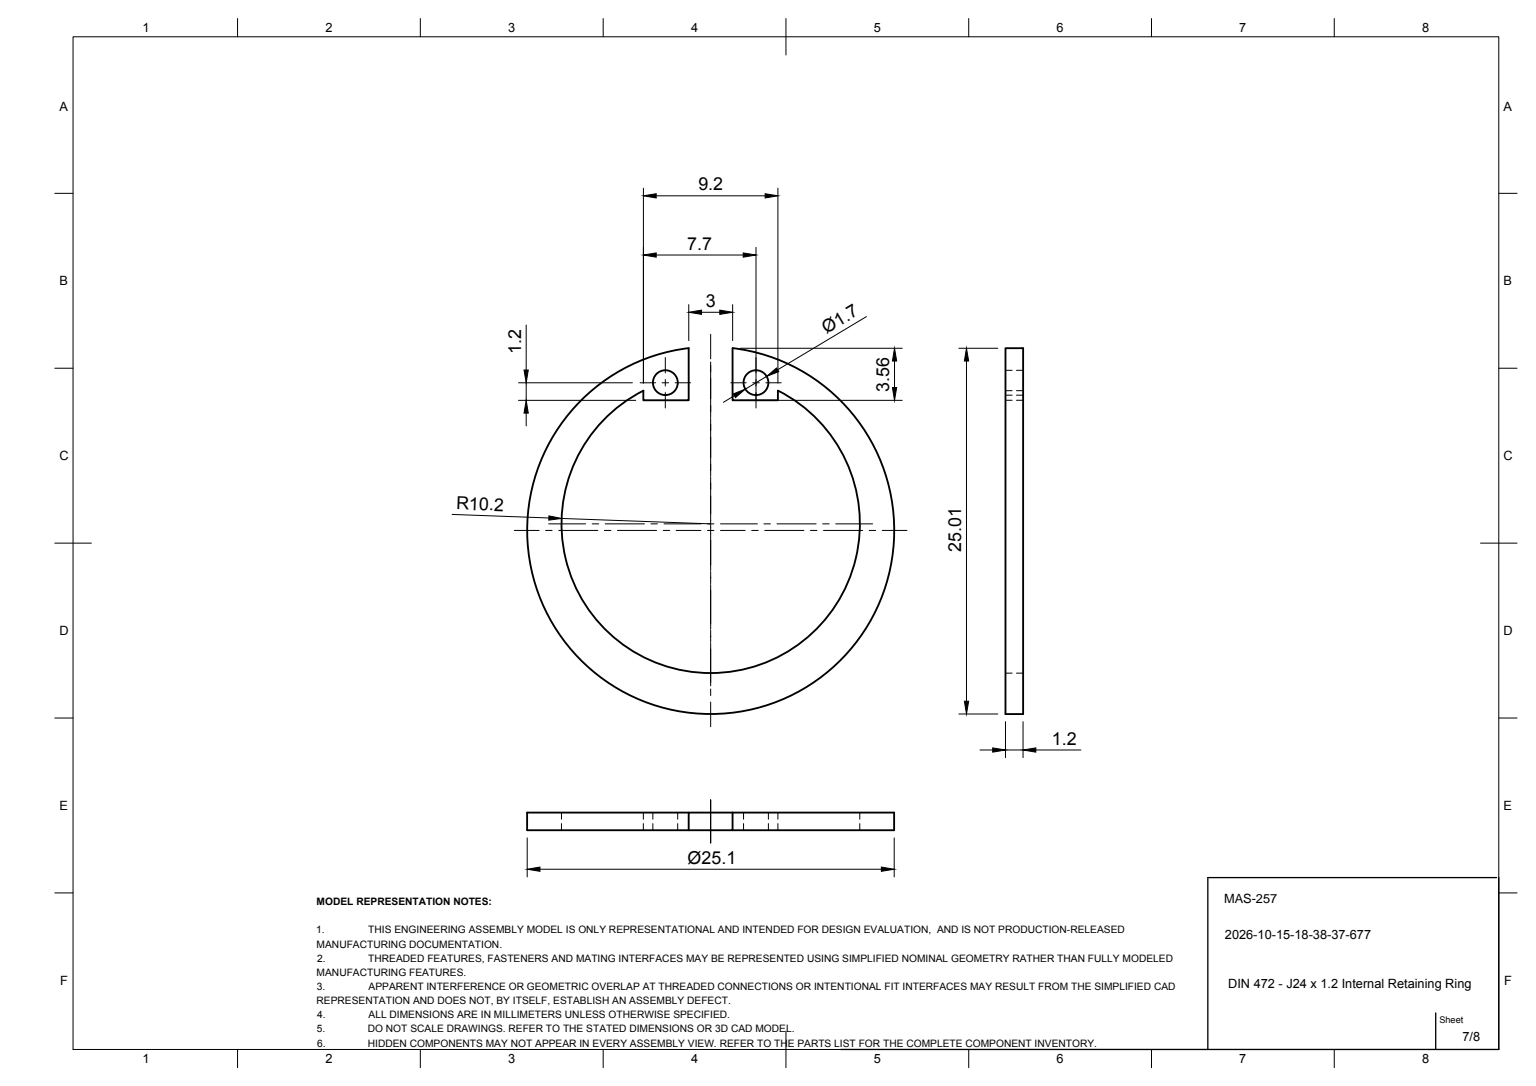
ISO-10303-21;
HEADER;
FILE_DESCRIPTION((''),'2;1');
FILE_NAME('DIN 472 - J24 x 1.2 Internal Retaining Ring.step','2026-10-05T22:33:56+05:00',(''),(''),'','','');
FILE_SCHEMA (('AUTOMOTIVE_DESIGN { 1 0 10303 214 3 1 1 }'));
ENDSEC;
DATA;
#10=MECHANICAL_DESIGN_GEOMETRIC_PRESENTATION_REPRESENTATION('',(#435),#16942);
#421=SHAPE_REPRESENTATION_RELATIONSHIP('SRR','None',#17025,#428) ;
#428=ADVANCED_BREP_SHAPE_REPRESENTATION('',(#442),#16941) ;
#435=STYLED_ITEM('',(#17069),#442) ;
#442=MANIFOLD_SOLID_BREP('DIN 472 - J24 x 1.2 Internal Retaining Ring',
#8184) ;
#733=FACE_BOUND('',#1985,.T.) ;
#734=FACE_BOUND('',#1986,.T.) ;
#735=FACE_BOUND('',#1994,.T.) ;
#736=FACE_BOUND('',#1995,.T.) ;
#969=PLANE('',#8900) ;
#970=PLANE('',#8901) ;
#971=PLANE('',#8902) ;
#972=PLANE('',#8903) ;
#973=PLANE('',#8909) ;
#974=PLANE('',#8910) ;
#975=PLANE('',#8913) ;
#976=PLANE('',#8916) ;
#1057=CYLINDRICAL_SURFACE('',#8897,0.85) ;
#1058=CYLINDRICAL_SURFACE('',#8907,0.85) ;
#1059=CYLINDRICAL_SURFACE('',#8911,10.2) ;
#1060=CYLINDRICAL_SURFACE('',#8914,12.55) ;
#1491=FACE_OUTER_BOUND('',#1980,.T.) ;
#1492=FACE_OUTER_BOUND('',#1981,.T.) ;
#1493=FACE_OUTER_BOUND('',#1982,.T.) ;
#1494=FACE_OUTER_BOUND('',#1983,.T.) ;
#1495=FACE_OUTER_BOUND('',#1984,.T.) ;
#1496=FACE_OUTER_BOUND('',#1987,.T.) ;
#1497=FACE_OUTER_BOUND('',#1988,.T.) ;
#1498=FACE_OUTER_BOUND('',#1989,.T.) ;
#1499=FACE_OUTER_BOUND('',#1990,.T.) ;
#1500=FACE_OUTER_BOUND('',#1991,.T.) ;
#1501=FACE_OUTER_BOUND('',#1992,.T.) ;
#1502=FACE_OUTER_BOUND('',#1993,.T.) ;
#1980=EDGE_LOOP('',(#7647,#7648,#7649,#7650)) ;
#1981=EDGE_LOOP('',(#7651,#7652,#7653,#7654)) ;
#1982=EDGE_LOOP('',(#7655,#7656,#7657,#7658)) ;
#1983=EDGE_LOOP('',(#7659,#7660,#7661,#7662)) ;
#1984=EDGE_LOOP('',(#7663,#7664,#7665,#7666,#7667,#7668,#7669,#7670)) ;
#1985=EDGE_LOOP('',(#7671)) ;
#1986=EDGE_LOOP('',(#7672)) ;
#1987=EDGE_LOOP('',(#7673,#7674,#7675,#7676)) ;
#1988=EDGE_LOOP('',(#7677,#7678,#7679,#7680)) ;
#1989=EDGE_LOOP('',(#7681,#7682,#7683,#7684)) ;
#1990=EDGE_LOOP('',(#7685,#7686,#7687,#7688)) ;
#1991=EDGE_LOOP('',(#7689,#7690,#7691,#7692)) ;
#1992=EDGE_LOOP('',(#7693,#7694,#7695,#7696)) ;
#1993=EDGE_LOOP('',(#7697,#7698,#7699,#7700,#7701,#7702,#7703,#7704)) ;
#1994=EDGE_LOOP('',(#7705)) ;
#1995=EDGE_LOOP('',(#7706)) ;
#2536=LINE('',#16812,#3098) ;
#2537=LINE('',#16817,#3099) ;
#2538=LINE('',#16819,#3100) ;
#2539=LINE('',#16821,#3101) ;
#2540=LINE('',#16822,#3102) ;
#2541=LINE('',#16825,#3103) ;
#2542=LINE('',#16827,#3104) ;
#2543=LINE('',#16828,#3105) ;
#2544=LINE('',#16831,#3106) ;
#2545=LINE('',#16833,#3107) ;
#2546=LINE('',#16834,#3108) ;
#2547=LINE('',#16839,#3109) ;
#2548=LINE('',#16841,#3110) ;
#2549=LINE('',#16843,#3111) ;
#2550=LINE('',#16850,#3112) ;
#2551=LINE('',#16853,#3113) ;
#2552=LINE('',#16855,#3114) ;
#2553=LINE('',#16856,#3115) ;
#2554=LINE('',#16859,#3116) ;
#2555=LINE('',#16860,#3117) ;
#2556=LINE('',#16865,#3118) ;
#2557=LINE('',#16866,#3119) ;
#3098=VECTOR('',#10784,0.85) ;
#3099=VECTOR('',#10789,10.) ;
#3100=VECTOR('',#10790,10.) ;
#3101=VECTOR('',#10791,10.) ;
#3102=VECTOR('',#10792,10.) ;
#3103=VECTOR('',#10795,10.) ;
#3104=VECTOR('',#10796,10.) ;
#3105=VECTOR('',#10797,10.) ;
#3106=VECTOR('',#10800,10.) ;
#3107=VECTOR('',#10801,10.) ;
#3108=VECTOR('',#10802,10.) ;
#3109=VECTOR('',#10807,10.) ;
#3110=VECTOR('',#10808,10.) ;
#3111=VECTOR('',#10809,10.) ;
#3112=VECTOR('',#10818,0.85) ;
#3113=VECTOR('',#10821,10.) ;
#3114=VECTOR('',#10822,10.) ;
#3115=VECTOR('',#10823,10.) ;
#3116=VECTOR('',#10826,10.) ;
#3117=VECTOR('',#10827,10.) ;
#3118=VECTOR('',#10834,10.) ;
#3119=VECTOR('',#10835,10.) ;
#3390=CIRCLE('',#8898,0.85) ;
#3391=CIRCLE('',#8899,0.85) ;
#3392=CIRCLE('',#8904,10.2) ;
#3393=CIRCLE('',#8905,12.55) ;
#3394=CIRCLE('',#8906,0.85) ;
#3395=CIRCLE('',#8908,0.85) ;
#3396=CIRCLE('',#8912,10.2) ;
#3397=CIRCLE('',#8915,12.55) ;
#4153=VERTEX_POINT('',#16809) ;
#4154=VERTEX_POINT('',#16811) ;
#4155=VERTEX_POINT('',#16815) ;
#4156=VERTEX_POINT('',#16816) ;
#4157=VERTEX_POINT('',#16818) ;
#4158=VERTEX_POINT('',#16820) ;
#4159=VERTEX_POINT('',#16824) ;
#4160=VERTEX_POINT('',#16826) ;
#4161=VERTEX_POINT('',#16830) ;
#4162=VERTEX_POINT('',#16832) ;
#4163=VERTEX_POINT('',#16836) ;
#4164=VERTEX_POINT('',#16838) ;
#4165=VERTEX_POINT('',#16840) ;
#4166=VERTEX_POINT('',#16842) ;
#4167=VERTEX_POINT('',#16845) ;
#4168=VERTEX_POINT('',#16848) ;
#4169=VERTEX_POINT('',#16852) ;
#4170=VERTEX_POINT('',#16854) ;
#4171=VERTEX_POINT('',#16858) ;
#4172=VERTEX_POINT('',#16864) ;
#5321=EDGE_CURVE('',#4153,#4153,#3390,.T.) ;
#5322=EDGE_CURVE('',#4153,#4154,#2536,.T.) ;
#5323=EDGE_CURVE('',#4154,#4154,#3391,.T.) ;
#5324=EDGE_CURVE('',#4155,#4156,#2537,.T.) ;
#5325=EDGE_CURVE('',#4157,#4155,#2538,.T.) ;
#5326=EDGE_CURVE('',#4158,#4157,#2539,.T.) ;
#5327=EDGE_CURVE('',#4156,#4158,#2540,.T.) ;
#5328=EDGE_CURVE('',#4158,#4159,#2541,.T.) ;
#5329=EDGE_CURVE('',#4160,#4157,#2542,.T.) ;
#5330=EDGE_CURVE('',#4159,#4160,#2543,.T.) ;
#5331=EDGE_CURVE('',#4161,#4160,#2544,.T.) ;
#5332=EDGE_CURVE('',#4162,#4161,#2545,.T.) ;
#5333=EDGE_CURVE('',#4159,#4162,#2546,.T.) ;
#5334=EDGE_CURVE('',#4155,#4163,#3392,.T.) ;
#5335=EDGE_CURVE('',#4163,#4164,#2547,.T.) ;
#5336=EDGE_CURVE('',#4164,#4165,#2548,.T.) ;
#5337=EDGE_CURVE('',#4165,#4166,#2549,.T.) ;
#5338=EDGE_CURVE('',#4166,#4161,#3393,.T.) ;
#5339=EDGE_CURVE('',#4167,#4167,#3394,.T.) ;
#5340=EDGE_CURVE('',#4168,#4168,#3395,.T.) ;
#5341=EDGE_CURVE('',#4168,#4167,#2550,.T.) ;
#5342=EDGE_CURVE('',#4169,#4163,#2551,.T.) ;
#5343=EDGE_CURVE('',#4169,#4170,#2552,.T.) ;
#5344=EDGE_CURVE('',#4170,#4164,#2553,.T.) ;
#5345=EDGE_CURVE('',#4170,#4171,#2554,.T.) ;
#5346=EDGE_CURVE('',#4171,#4165,#2555,.T.) ;
#5347=EDGE_CURVE('',#4156,#4169,#3396,.T.) ;
#5348=EDGE_CURVE('',#4172,#4171,#2556,.T.) ;
#5349=EDGE_CURVE('',#4166,#4172,#2557,.T.) ;
#5350=EDGE_CURVE('',#4172,#4162,#3397,.T.) ;
#7647=ORIENTED_EDGE('',*,*,#5321,.F.) ;
#7648=ORIENTED_EDGE('',*,*,#5322,.T.) ;
#7649=ORIENTED_EDGE('',*,*,#5323,.F.) ;
#7650=ORIENTED_EDGE('',*,*,#5322,.F.) ;
#7651=ORIENTED_EDGE('',*,*,#5324,.F.) ;
#7652=ORIENTED_EDGE('',*,*,#5325,.F.) ;
#7653=ORIENTED_EDGE('',*,*,#5326,.F.) ;
#7654=ORIENTED_EDGE('',*,*,#5327,.F.) ;
#7655=ORIENTED_EDGE('',*,*,#5328,.F.) ;
#7656=ORIENTED_EDGE('',*,*,#5326,.T.) ;
#7657=ORIENTED_EDGE('',*,*,#5329,.F.) ;
#7658=ORIENTED_EDGE('',*,*,#5330,.F.) ;
#7659=ORIENTED_EDGE('',*,*,#5331,.F.) ;
#7660=ORIENTED_EDGE('',*,*,#5332,.F.) ;
#7661=ORIENTED_EDGE('',*,*,#5333,.F.) ;
#7662=ORIENTED_EDGE('',*,*,#5330,.T.) ;
#7663=ORIENTED_EDGE('',*,*,#5331,.T.) ;
#7664=ORIENTED_EDGE('',*,*,#5329,.T.) ;
#7665=ORIENTED_EDGE('',*,*,#5325,.T.) ;
#7666=ORIENTED_EDGE('',*,*,#5334,.T.) ;
#7667=ORIENTED_EDGE('',*,*,#5335,.T.) ;
#7668=ORIENTED_EDGE('',*,*,#5336,.T.) ;
#7669=ORIENTED_EDGE('',*,*,#5337,.T.) ;
#7670=ORIENTED_EDGE('',*,*,#5338,.T.) ;
#7671=ORIENTED_EDGE('',*,*,#5323,.T.) ;
#7672=ORIENTED_EDGE('',*,*,#5339,.T.) ;
#7673=ORIENTED_EDGE('',*,*,#5340,.F.) ;
#7674=ORIENTED_EDGE('',*,*,#5341,.T.) ;
#7675=ORIENTED_EDGE('',*,*,#5339,.F.) ;
#7676=ORIENTED_EDGE('',*,*,#5341,.F.) ;
#7677=ORIENTED_EDGE('',*,*,#5342,.F.) ;
#7678=ORIENTED_EDGE('',*,*,#5343,.T.) ;
#7679=ORIENTED_EDGE('',*,*,#5344,.T.) ;
#7680=ORIENTED_EDGE('',*,*,#5335,.F.) ;
#7681=ORIENTED_EDGE('',*,*,#5345,.T.) ;
#7682=ORIENTED_EDGE('',*,*,#5346,.T.) ;
#7683=ORIENTED_EDGE('',*,*,#5336,.F.) ;
#7684=ORIENTED_EDGE('',*,*,#5344,.F.) ;
#7685=ORIENTED_EDGE('',*,*,#5324,.T.) ;
#7686=ORIENTED_EDGE('',*,*,#5347,.T.) ;
#7687=ORIENTED_EDGE('',*,*,#5342,.T.) ;
#7688=ORIENTED_EDGE('',*,*,#5334,.F.) ;
#7689=ORIENTED_EDGE('',*,*,#5348,.F.) ;
#7690=ORIENTED_EDGE('',*,*,#5349,.F.) ;
#7691=ORIENTED_EDGE('',*,*,#5337,.F.) ;
#7692=ORIENTED_EDGE('',*,*,#5346,.F.) ;
#7693=ORIENTED_EDGE('',*,*,#5349,.T.) ;
#7694=ORIENTED_EDGE('',*,*,#5350,.T.) ;
#7695=ORIENTED_EDGE('',*,*,#5332,.T.) ;
#7696=ORIENTED_EDGE('',*,*,#5338,.F.) ;
#7697=ORIENTED_EDGE('',*,*,#5333,.T.) ;
#7698=ORIENTED_EDGE('',*,*,#5350,.F.) ;
#7699=ORIENTED_EDGE('',*,*,#5348,.T.) ;
#7700=ORIENTED_EDGE('',*,*,#5345,.F.) ;
#7701=ORIENTED_EDGE('',*,*,#5343,.F.) ;
#7702=ORIENTED_EDGE('',*,*,#5347,.F.) ;
#7703=ORIENTED_EDGE('',*,*,#5327,.T.) ;
#7704=ORIENTED_EDGE('',*,*,#5328,.T.) ;
#7705=ORIENTED_EDGE('',*,*,#5321,.T.) ;
#7706=ORIENTED_EDGE('',*,*,#5340,.T.) ;
#8166=ADVANCED_FACE('',(#1491),#1057,.F.) ;
#8167=ADVANCED_FACE('',(#1492),#969,.T.) ;
#8168=ADVANCED_FACE('',(#1493),#970,.T.) ;
#8169=ADVANCED_FACE('',(#1494),#971,.F.) ;
#8170=ADVANCED_FACE('',(#1495,#733,#734),#972,.T.) ;
#8171=ADVANCED_FACE('',(#1496),#1058,.F.) ;
#8172=ADVANCED_FACE('',(#1497),#973,.T.) ;
#8173=ADVANCED_FACE('',(#1498),#974,.T.) ;
#8174=ADVANCED_FACE('',(#1499),#1059,.F.) ;
#8175=ADVANCED_FACE('',(#1500),#975,.F.) ;
#8176=ADVANCED_FACE('',(#1501),#1060,.T.) ;
#8177=ADVANCED_FACE('',(#1502,#735,#736),#976,.F.) ;
#8184=CLOSED_SHELL('',(#8166,#8167,#8168,#8169,#8170,#8171,#8172,#8173,
#8174,#8175,#8176,#8177)) ;
#8896=AXIS2_PLACEMENT_3D('',#16807,#10778,#10779) ;
#8897=AXIS2_PLACEMENT_3D('',#16808,#10780,#10781) ;
#8898=AXIS2_PLACEMENT_3D('',#16810,#10782,#10783) ;
#8899=AXIS2_PLACEMENT_3D('',#16813,#10785,#10786) ;
#8900=AXIS2_PLACEMENT_3D('',#16814,#10787,#10788) ;
#8901=AXIS2_PLACEMENT_3D('',#16823,#10793,#10794) ;
#8902=AXIS2_PLACEMENT_3D('',#16829,#10798,#10799) ;
#8903=AXIS2_PLACEMENT_3D('',#16835,#10803,#10804) ;
#8904=AXIS2_PLACEMENT_3D('',#16837,#10805,#10806) ;
#8905=AXIS2_PLACEMENT_3D('',#16844,#10810,#10811) ;
#8906=AXIS2_PLACEMENT_3D('',#16846,#10812,#10813) ;
#8907=AXIS2_PLACEMENT_3D('',#16847,#10814,#10815) ;
#8908=AXIS2_PLACEMENT_3D('',#16849,#10816,#10817) ;
#8909=AXIS2_PLACEMENT_3D('',#16851,#10819,#10820) ;
#8910=AXIS2_PLACEMENT_3D('',#16857,#10824,#10825) ;
#8911=AXIS2_PLACEMENT_3D('',#16861,#10828,#10829) ;
#8912=AXIS2_PLACEMENT_3D('',#16862,#10830,#10831) ;
#8913=AXIS2_PLACEMENT_3D('',#16863,#10832,#10833) ;
#8914=AXIS2_PLACEMENT_3D('',#16867,#10836,#10837) ;
#8915=AXIS2_PLACEMENT_3D('',#16868,#10838,#10839) ;
#8916=AXIS2_PLACEMENT_3D('',#16869,#10840,#10841) ;
#10778=DIRECTION('axis',(0.,0.,1.)) ;
#10779=DIRECTION('refdir',(1.,0.,0.)) ;
#10780=DIRECTION('center_axis',(1.,0.,0.)) ;
#10781=DIRECTION('ref_axis',(0.,0.,-1.)) ;
#10782=DIRECTION('center_axis',(1.,0.,0.)) ;
#10783=DIRECTION('ref_axis',(0.,0.,-1.)) ;
#10784=DIRECTION('',(1.,0.,0.)) ;
#10785=DIRECTION('center_axis',(-1.,0.,0.)) ;
#10786=DIRECTION('ref_axis',(0.,0.,-1.)) ;
#10787=DIRECTION('center_axis',(0.,0.,-1.)) ;
#10788=DIRECTION('ref_axis',(0.,1.,0.)) ;
#10789=DIRECTION('',(-1.,0.,0.)) ;
#10790=DIRECTION('',(0.,1.,0.)) ;
#10791=DIRECTION('',(1.,0.,0.)) ;
#10792=DIRECTION('',(0.,-1.,0.)) ;
#10793=DIRECTION('center_axis',(0.,-1.,0.)) ;
#10794=DIRECTION('ref_axis',(0.,0.,-1.)) ;
#10795=DIRECTION('',(0.,0.,1.)) ;
#10796=DIRECTION('',(0.,0.,-1.)) ;
#10797=DIRECTION('',(1.,0.,0.)) ;
#10798=DIRECTION('center_axis',(0.,0.,-1.)) ;
#10799=DIRECTION('ref_axis',(0.,1.,0.)) ;
#10800=DIRECTION('',(0.,-1.,0.)) ;
#10801=DIRECTION('',(1.,0.,0.)) ;
#10802=DIRECTION('',(0.,1.,0.)) ;
#10803=DIRECTION('center_axis',(1.,0.,0.)) ;
#10804=DIRECTION('ref_axis',(0.,0.,-1.)) ;
#10805=DIRECTION('center_axis',(-1.,0.,0.)) ;
#10806=DIRECTION('ref_axis',(0.,0.,-1.)) ;
#10807=DIRECTION('',(0.,-1.,0.)) ;
#10808=DIRECTION('',(0.,0.,-1.)) ;
#10809=DIRECTION('',(0.,1.,0.)) ;
#10810=DIRECTION('center_axis',(1.,0.,0.)) ;
#10811=DIRECTION('ref_axis',(0.,0.,-1.)) ;
#10812=DIRECTION('center_axis',(-1.,0.,0.)) ;
#10813=DIRECTION('ref_axis',(0.,0.,-1.)) ;
#10814=DIRECTION('center_axis',(1.,0.,0.)) ;
#10815=DIRECTION('ref_axis',(0.,0.,-1.)) ;
#10816=DIRECTION('center_axis',(1.,0.,0.)) ;
#10817=DIRECTION('ref_axis',(0.,0.,-1.)) ;
#10818=DIRECTION('',(1.,0.,0.)) ;
#10819=DIRECTION('center_axis',(0.,0.,1.)) ;
#10820=DIRECTION('ref_axis',(0.,-1.,0.)) ;
#10821=DIRECTION('',(1.,0.,0.)) ;
#10822=DIRECTION('',(0.,-1.,0.)) ;
#10823=DIRECTION('',(1.,0.,0.)) ;
#10824=DIRECTION('center_axis',(0.,-1.,0.)) ;
#10825=DIRECTION('ref_axis',(0.,0.,-1.)) ;
#10826=DIRECTION('',(0.,0.,-1.)) ;
#10827=DIRECTION('',(1.,0.,0.)) ;
#10828=DIRECTION('center_axis',(1.,0.,0.)) ;
#10829=DIRECTION('ref_axis',(0.,-1.,-6.12323399573677E-17)) ;
#10830=DIRECTION('center_axis',(-1.,0.,0.)) ;
#10831=DIRECTION('ref_axis',(0.,0.,-1.)) ;
#10832=DIRECTION('center_axis',(0.,0.,1.)) ;
#10833=DIRECTION('ref_axis',(0.,-1.,0.)) ;
#10834=DIRECTION('',(0.,-1.,0.)) ;
#10835=DIRECTION('',(-1.,0.,0.)) ;
#10836=DIRECTION('center_axis',(1.,0.,0.)) ;
#10837=DIRECTION('ref_axis',(0.,-1.,1.83697019872103E-16)) ;
#10838=DIRECTION('center_axis',(1.,0.,0.)) ;
#10839=DIRECTION('ref_axis',(0.,0.,-1.)) ;
#10840=DIRECTION('center_axis',(1.,0.,0.)) ;
#10841=DIRECTION('ref_axis',(0.,0.,-1.)) ;
#16807=CARTESIAN_POINT('',(0.,0.,0.)) ;
#16808=CARTESIAN_POINT('Origin',(27.85,35.6,22.4)) ;
#16809=CARTESIAN_POINT('',(27.85,35.6,23.25)) ;
#16810=CARTESIAN_POINT('Origin',(27.85,35.6,22.4)) ;
#16811=CARTESIAN_POINT('',(29.05,35.6,23.25)) ;
#16812=CARTESIAN_POINT('',(27.85,35.6,23.25)) ;
#16813=CARTESIAN_POINT('Origin',(29.05,35.6,22.4)) ;
#16814=CARTESIAN_POINT('Origin',(27.85,34.4,20.9)) ;
#16815=CARTESIAN_POINT('',(29.05,35.0538453413928,20.9)) ;
#16816=CARTESIAN_POINT('',(27.85,35.0538453413928,20.9)) ;
#16817=CARTESIAN_POINT('',(27.85,35.0538453413928,20.9)) ;
#16818=CARTESIAN_POINT('',(29.05,34.4,20.9)) ;
#16819=CARTESIAN_POINT('',(29.05,36.4,20.9)) ;
#16820=CARTESIAN_POINT('',(27.85,34.4,20.9)) ;
#16821=CARTESIAN_POINT('',(27.85,34.4,20.9)) ;
#16822=CARTESIAN_POINT('',(27.85,36.4,20.9)) ;
#16823=CARTESIAN_POINT('Origin',(27.85,34.4,24.)) ;
#16824=CARTESIAN_POINT('',(27.85,34.4,24.)) ;
#16825=CARTESIAN_POINT('',(27.85,34.4,20.9)) ;
#16826=CARTESIAN_POINT('',(29.05,34.4,24.)) ;
#16827=CARTESIAN_POINT('',(29.05,34.4,20.9)) ;
#16828=CARTESIAN_POINT('',(27.85,34.4,24.)) ;
#16829=CARTESIAN_POINT('Origin',(27.85,34.5,24.)) ;
#16830=CARTESIAN_POINT('',(29.05,37.9600361155175,24.)) ;
#16831=CARTESIAN_POINT('',(29.05,34.4,24.)) ;
#16832=CARTESIAN_POINT('',(27.85,37.9600361155175,24.)) ;
#16833=CARTESIAN_POINT('',(27.85,37.9600361155175,24.)) ;
#16834=CARTESIAN_POINT('',(27.85,30.,24.)) ;
#16835=CARTESIAN_POINT('Origin',(29.05,25.5,25.5)) ;
#16836=CARTESIAN_POINT('',(29.05,35.0538453413928,30.1)) ;
#16837=CARTESIAN_POINT('Origin',(29.05,25.95,25.5)) ;
#16838=CARTESIAN_POINT('',(29.05,34.4,30.1)) ;
#16839=CARTESIAN_POINT('',(29.05,36.4,30.1)) ;
#16840=CARTESIAN_POINT('',(29.05,34.4,27.)) ;
#16841=CARTESIAN_POINT('',(29.05,34.4,30.1)) ;
#16842=CARTESIAN_POINT('',(29.05,37.9600361155175,27.)) ;
#16843=CARTESIAN_POINT('',(29.05,32.,27.)) ;
#16844=CARTESIAN_POINT('Origin',(29.05,25.5,25.5)) ;
#16845=CARTESIAN_POINT('',(29.05,35.6,29.45)) ;
#16846=CARTESIAN_POINT('Origin',(29.05,35.6,28.6)) ;
#16847=CARTESIAN_POINT('Origin',(27.85,35.6,28.6)) ;
#16848=CARTESIAN_POINT('',(27.85,35.6,29.45)) ;
#16849=CARTESIAN_POINT('Origin',(27.85,35.6,28.6)) ;
#16850=CARTESIAN_POINT('',(27.85,35.6,29.45)) ;
#16851=CARTESIAN_POINT('Origin',(27.85,36.4,30.1)) ;
#16852=CARTESIAN_POINT('',(27.85,35.0538453413928,30.1)) ;
#16853=CARTESIAN_POINT('',(27.85,35.0538453413928,30.1)) ;
#16854=CARTESIAN_POINT('',(27.85,34.4,30.1)) ;
#16855=CARTESIAN_POINT('',(27.85,36.4,30.1)) ;
#16856=CARTESIAN_POINT('',(27.85,34.4,30.1)) ;
#16857=CARTESIAN_POINT('Origin',(27.85,34.4,30.1)) ;
#16858=CARTESIAN_POINT('',(27.85,34.4,27.)) ;
#16859=CARTESIAN_POINT('',(27.85,34.4,30.1)) ;
#16860=CARTESIAN_POINT('',(27.85,34.4,27.)) ;
#16861=CARTESIAN_POINT('Origin',(27.85,25.95,25.5)) ;
#16862=CARTESIAN_POINT('Origin',(27.85,25.95,25.5)) ;
#16863=CARTESIAN_POINT('Origin',(27.85,38.5,27.)) ;
#16864=CARTESIAN_POINT('',(27.85,37.9600361155175,27.)) ;
#16865=CARTESIAN_POINT('',(27.85,32.,27.)) ;
#16866=CARTESIAN_POINT('',(27.85,37.9600361155175,27.)) ;
#16867=CARTESIAN_POINT('Origin',(27.85,25.5,25.5)) ;
#16868=CARTESIAN_POINT('Origin',(27.85,25.5,25.5)) ;
#16869=CARTESIAN_POINT('Origin',(27.85,25.5,25.5)) ;
#16932=UNCERTAINTY_MEASURE_WITH_UNIT(LENGTH_MEASURE(0.01),#16943,
'DISTANCE_ACCURACY_VALUE',
'Maximum model space distance between geometric entities at asserted c
onnectivities') ;
#16933=UNCERTAINTY_MEASURE_WITH_UNIT(LENGTH_MEASURE(0.01),#16943,
'DISTANCE_ACCURACY_VALUE',
'Maximum model space distance between geometric entities at asserted c
onnectivities') ;
#16941=(
GEOMETRIC_REPRESENTATION_CONTEXT(3)
GLOBAL_UNCERTAINTY_ASSIGNED_CONTEXT((#16932))
GLOBAL_UNIT_ASSIGNED_CONTEXT((#16943,#16945,#16946))
REPRESENTATION_CONTEXT('','3D')
) ;
#16942=(
GEOMETRIC_REPRESENTATION_CONTEXT(3)
GLOBAL_UNCERTAINTY_ASSIGNED_CONTEXT((#16933))
GLOBAL_UNIT_ASSIGNED_CONTEXT((#16943,#16945,#16946))
REPRESENTATION_CONTEXT('','3D')
) ;
#16943=(
LENGTH_UNIT()
NAMED_UNIT(*)
SI_UNIT(.MILLI.,.METRE.)
) ;
#16945=(
NAMED_UNIT(*)
PLANE_ANGLE_UNIT()
SI_UNIT($,.RADIAN.)
) ;
#16946=(
NAMED_UNIT(*)
SI_UNIT($,.STERADIAN.)
SOLID_ANGLE_UNIT()
) ;
#16954=SHAPE_DEFINITION_REPRESENTATION(#16962,#17025) ;
#16962=PRODUCT_DEFINITION_SHAPE('',$,#17034) ;
#17025=SHAPE_REPRESENTATION('',(#8896),#16941) ;
#17026=PRODUCT_DEFINITION_CONTEXT('part definition',#17052,'design') ;
#17034=PRODUCT_DEFINITION('DIN 472 - J24 x 1.2 Internal Retaining Ring',
'DIN 472 - J24 x 1.2 Internal Retaining Ring',#17042,#17026) ;
#17042=PRODUCT_DEFINITION_FORMATION('',$,#17061) ;
#17052=APPLICATION_CONTEXT(
'Core Data for Automotive Mechanical Design Process') ;
#17053=PRODUCT_CONTEXT('part definition',#17052,'mechanical') ;
#17061=PRODUCT('DIN 472 - J24 x 1.2 Internal Retaining Ring',
'DIN 472 - J24 x 1.2 Internal Retaining Ring',$,(#17053)) ;
#17069=PRESENTATION_STYLE_ASSIGNMENT((#17077)) ;
#17077=SURFACE_STYLE_USAGE(.BOTH.,#17085) ;
#17085=SURFACE_SIDE_STYLE('',(#17093)) ;
#17093=SURFACE_STYLE_FILL_AREA(#17101) ;
#17101=FILL_AREA_STYLE(
'MAS-257 Metallic Sheet - DIN 472 - J24 x 1.2 Internal Retaining R',(#17109)) ;
#17109=FILL_AREA_STYLE_COLOUR(
'MAS-257 Metallic Sheet - DIN 472 - J24 x 1.2 Internal Retaining R',#17117) ;
#17117=COLOUR_RGB(
'MAS-257 Metallic Sheet - DIN 472 - J24 x 1.2 Internal Retaining R', 0.66274510, 0.83137255, 0.94901961) ;
ENDSEC;
END-ISO-10303-21;
